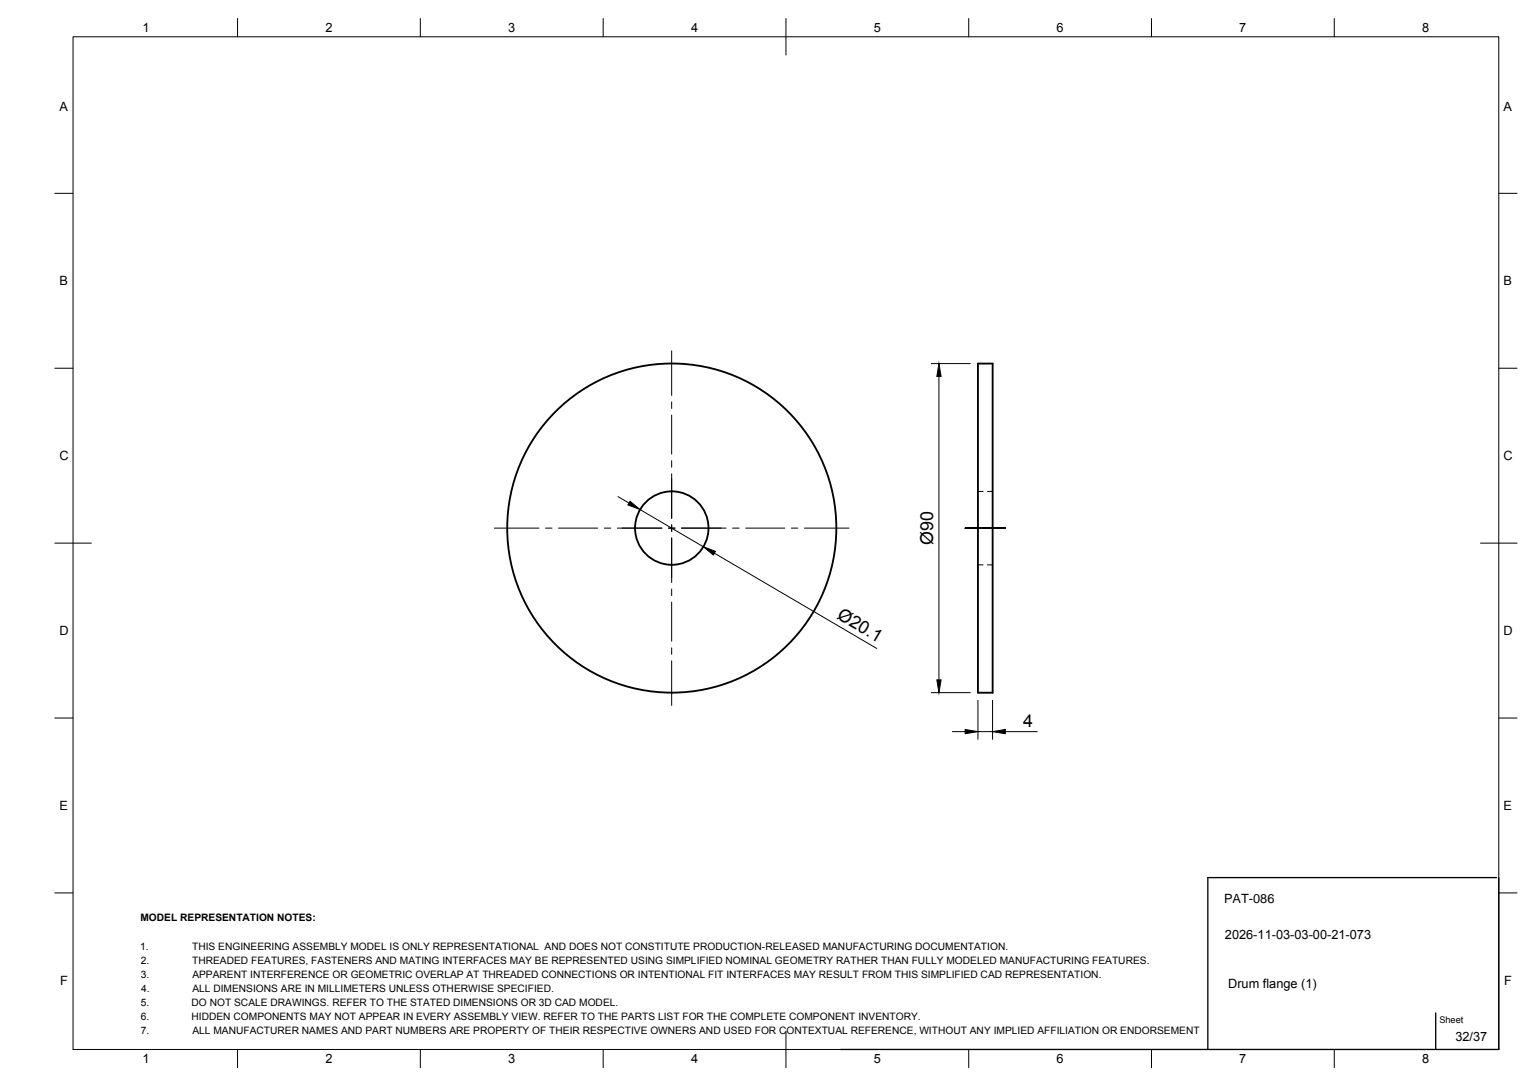
ISO-10303-21;
HEADER;
/* Generated by software containing ST-Developer
 * from STEP Tools, Inc. (www.steptools.com) 
 */

FILE_DESCRIPTION(
/* description */ ('Ratchet and pawl hand winch drum'),
/* implementation_level */ '2;1');

FILE_NAME(
/* name */ 'Drum flange (1).step',
/* time_stamp */ '2026-10-27T12:42:58-07:00',
/* author */ (''),
/* organization */ (''),
/* preprocessor_version */ 'ST-DEVELOPER v20.2',
/* originating_system */ 'Autodesk Translation Framework v15.17.0.0',
/* authorisation */ '');

FILE_SCHEMA (('AUTOMOTIVE_DESIGN { 1 0 10303 214 3 1 1 }'));
ENDSEC;

DATA;
#10=MECHANICAL_DESIGN_GEOMETRIC_PRESENTATION_REPRESENTATION('',(#416),#11801);
#347=SHAPE_REPRESENTATION_RELATIONSHIP('SRR','None',#11975,#381);
#381=ADVANCED_BREP_SHAPE_REPRESENTATION('',(#449),#11792);
#416=STYLED_ITEM('',(#12199),#449);
#449=MANIFOLD_SOLID_BREP('Body1',#6295);
#580=FACE_BOUND('',#1558,.T.);
#581=FACE_BOUND('',#1560,.T.);
#744=PLANE('',#7126);
#745=PLANE('',#7127);
#1075=FACE_OUTER_BOUND('',#1555,.T.);
#1076=FACE_OUTER_BOUND('',#1556,.T.);
#1077=FACE_OUTER_BOUND('',#1557,.T.);
#1078=FACE_OUTER_BOUND('',#1559,.T.);
#1555=EDGE_LOOP('',(#5227,#5228,#5229,#5230));
#1556=EDGE_LOOP('',(#5231,#5232,#5233,#5234));
#1557=EDGE_LOOP('',(#5235));
#1558=EDGE_LOOP('',(#5236));
#1559=EDGE_LOOP('',(#5237));
#1560=EDGE_LOOP('',(#5238));
#1978=LINE('',#10910,#2489);
#1979=LINE('',#10916,#2490);
#2489=VECTOR('',#8525,1.005);
#2490=VECTOR('',#8532,4.5);
#2892=CIRCLE('',#7121,1.005);
#2893=CIRCLE('',#7122,1.005);
#2894=CIRCLE('',#7124,4.5);
#2895=CIRCLE('',#7125,4.5);
#3275=VERTEX_POINT('',#10907);
#3276=VERTEX_POINT('',#10909);
#3277=VERTEX_POINT('',#10913);
#3278=VERTEX_POINT('',#10915);
#3957=EDGE_CURVE('',#3275,#3275,#2892,.T.);
#3958=EDGE_CURVE('',#3275,#3276,#1978,.T.);
#3959=EDGE_CURVE('',#3276,#3276,#2893,.T.);
#3960=EDGE_CURVE('',#3277,#3277,#2894,.T.);
#3961=EDGE_CURVE('',#3277,#3278,#1979,.T.);
#3962=EDGE_CURVE('',#3278,#3278,#2895,.T.);
#5227=ORIENTED_EDGE('',*,*,#3957,.F.);
#5228=ORIENTED_EDGE('',*,*,#3958,.T.);
#5229=ORIENTED_EDGE('',*,*,#3959,.T.);
#5230=ORIENTED_EDGE('',*,*,#3958,.F.);
#5231=ORIENTED_EDGE('',*,*,#3960,.F.);
#5232=ORIENTED_EDGE('',*,*,#3961,.T.);
#5233=ORIENTED_EDGE('',*,*,#3962,.T.);
#5234=ORIENTED_EDGE('',*,*,#3961,.F.);
#5235=ORIENTED_EDGE('',*,*,#3960,.T.);
#5236=ORIENTED_EDGE('',*,*,#3957,.T.);
#5237=ORIENTED_EDGE('',*,*,#3962,.F.);
#5238=ORIENTED_EDGE('',*,*,#3959,.F.);
#5891=CYLINDRICAL_SURFACE('',#7120,1.005);
#5892=CYLINDRICAL_SURFACE('',#7123,4.5);
#6145=ADVANCED_FACE('',(#1075),#5891,.F.);
#6146=ADVANCED_FACE('',(#1076),#5892,.T.);
#6147=ADVANCED_FACE('',(#1077,#580),#744,.T.);
#6148=ADVANCED_FACE('',(#1078,#581),#745,.F.);
#6295=CLOSED_SHELL('',(#6145,#6146,#6147,#6148));
#7119=AXIS2_PLACEMENT_3D('',#10905,#8519,#8520);
#7120=AXIS2_PLACEMENT_3D('',#10906,#8521,#8522);
#7121=AXIS2_PLACEMENT_3D('',#10908,#8523,#8524);
#7122=AXIS2_PLACEMENT_3D('',#10911,#8526,#8527);
#7123=AXIS2_PLACEMENT_3D('',#10912,#8528,#8529);
#7124=AXIS2_PLACEMENT_3D('',#10914,#8530,#8531);
#7125=AXIS2_PLACEMENT_3D('',#10917,#8533,#8534);
#7126=AXIS2_PLACEMENT_3D('',#10918,#8535,#8536);
#7127=AXIS2_PLACEMENT_3D('',#10919,#8537,#8538);
#8519=DIRECTION('axis',(0.,0.,1.));
#8520=DIRECTION('refdir',(1.,0.,0.));
#8521=DIRECTION('center_axis',(0.,1.,0.));
#8522=DIRECTION('ref_axis',(1.,0.,0.));
#8523=DIRECTION('center_axis',(0.,-1.,0.));
#8524=DIRECTION('ref_axis',(1.,0.,0.));
#8525=DIRECTION('',(0.,-1.,0.));
#8526=DIRECTION('center_axis',(0.,-1.,0.));
#8527=DIRECTION('ref_axis',(1.,0.,0.));
#8528=DIRECTION('center_axis',(0.,1.,0.));
#8529=DIRECTION('ref_axis',(1.,0.,0.));
#8530=DIRECTION('center_axis',(0.,1.,0.));
#8531=DIRECTION('ref_axis',(1.,0.,0.));
#8532=DIRECTION('',(0.,-1.,0.));
#8533=DIRECTION('center_axis',(0.,1.,0.));
#8534=DIRECTION('ref_axis',(1.,0.,0.));
#8535=DIRECTION('center_axis',(0.,1.,0.));
#8536=DIRECTION('ref_axis',(1.,0.,0.));
#8537=DIRECTION('center_axis',(0.,1.,0.));
#8538=DIRECTION('ref_axis',(1.,0.,0.));
#10905=CARTESIAN_POINT('',(0.,0.,0.));
#10906=CARTESIAN_POINT('Origin',(0.,13.,6.53));
#10907=CARTESIAN_POINT('',(-1.005,13.4,6.53));
#10908=CARTESIAN_POINT('Origin',(0.,13.4,6.53));
#10909=CARTESIAN_POINT('',(-1.005,13.,6.53));
#10910=CARTESIAN_POINT('',(-1.005,13.,6.53));
#10911=CARTESIAN_POINT('Origin',(0.,13.,6.53));
#10912=CARTESIAN_POINT('Origin',(0.,13.,6.53));
#10913=CARTESIAN_POINT('',(-4.5,13.4,6.53));
#10914=CARTESIAN_POINT('Origin',(0.,13.4,6.53));
#10915=CARTESIAN_POINT('',(-4.5,13.,6.53));
#10916=CARTESIAN_POINT('',(-4.5,13.,6.53));
#10917=CARTESIAN_POINT('Origin',(0.,13.,6.53));
#10918=CARTESIAN_POINT('Origin',(0.,13.4,6.53));
#10919=CARTESIAN_POINT('Origin',(0.,13.,6.53));
#11752=UNCERTAINTY_MEASURE_WITH_UNIT(LENGTH_MEASURE(0.001),#11802,
'DISTANCE_ACCURACY_VALUE',
'Maximum model space distance between geometric entities at asserted c
onnectivities');
#11761=UNCERTAINTY_MEASURE_WITH_UNIT(LENGTH_MEASURE(0.001),#11802,
'DISTANCE_ACCURACY_VALUE',
'Maximum model space distance between geometric entities at asserted c
onnectivities');
#11792=(
GEOMETRIC_REPRESENTATION_CONTEXT(3)
GLOBAL_UNCERTAINTY_ASSIGNED_CONTEXT((#11752))
GLOBAL_UNIT_ASSIGNED_CONTEXT((#11802,#11804,#11805))
REPRESENTATION_CONTEXT('','3D')
);
#11801=(
GEOMETRIC_REPRESENTATION_CONTEXT(3)
GLOBAL_UNCERTAINTY_ASSIGNED_CONTEXT((#11761))
GLOBAL_UNIT_ASSIGNED_CONTEXT((#11802,#11804,#11805))
REPRESENTATION_CONTEXT('','3D')
);
#11802=(
LENGTH_UNIT()
NAMED_UNIT(*)
SI_UNIT(.CENTI.,.METRE.)
);
#11804=(
NAMED_UNIT(*)
PLANE_ANGLE_UNIT()
SI_UNIT($,.RADIAN.)
);
#11805=(
NAMED_UNIT(*)
SI_UNIT($,.STERADIAN.)
SOLID_ANGLE_UNIT()
);
#11836=SHAPE_DEFINITION_REPRESENTATION(#11877,#11975);
#11877=PRODUCT_DEFINITION_SHAPE('',$,#12015);
#11975=SHAPE_REPRESENTATION('',(#7119),#11792);
#11984=PRODUCT_DEFINITION_CONTEXT('part definition',#12103,'design');
#12015=PRODUCT_DEFINITION('Drum flange (1)','Drum flange (1)',#12054,#11984);
#12054=PRODUCT_DEFINITION_FORMATION('',$,#12135);
#12103=APPLICATION_CONTEXT(
'Core Data for Automotive Mechanical Design Process');
#12104=PRODUCT_CONTEXT('part definition',#12103,'mechanical');
#12135=PRODUCT('Drum flange (1)','Drum flange (1)','Drum flange (1)',(#12104));
#12193=COLOUR_RGB('Light Blue',0.38,0.62,0.78);
#12194=FILL_AREA_STYLE_COLOUR('',#12193);
#12195=FILL_AREA_STYLE('',(#12194));
#12196=SURFACE_STYLE_FILL_AREA(#12195);
#12197=SURFACE_SIDE_STYLE('',(#12196));
#12198=SURFACE_STYLE_USAGE(.BOTH.,#12197);
#12199=PRESENTATION_STYLE_ASSIGNMENT((#12198));
ENDSEC;
END-ISO-10303-21;
